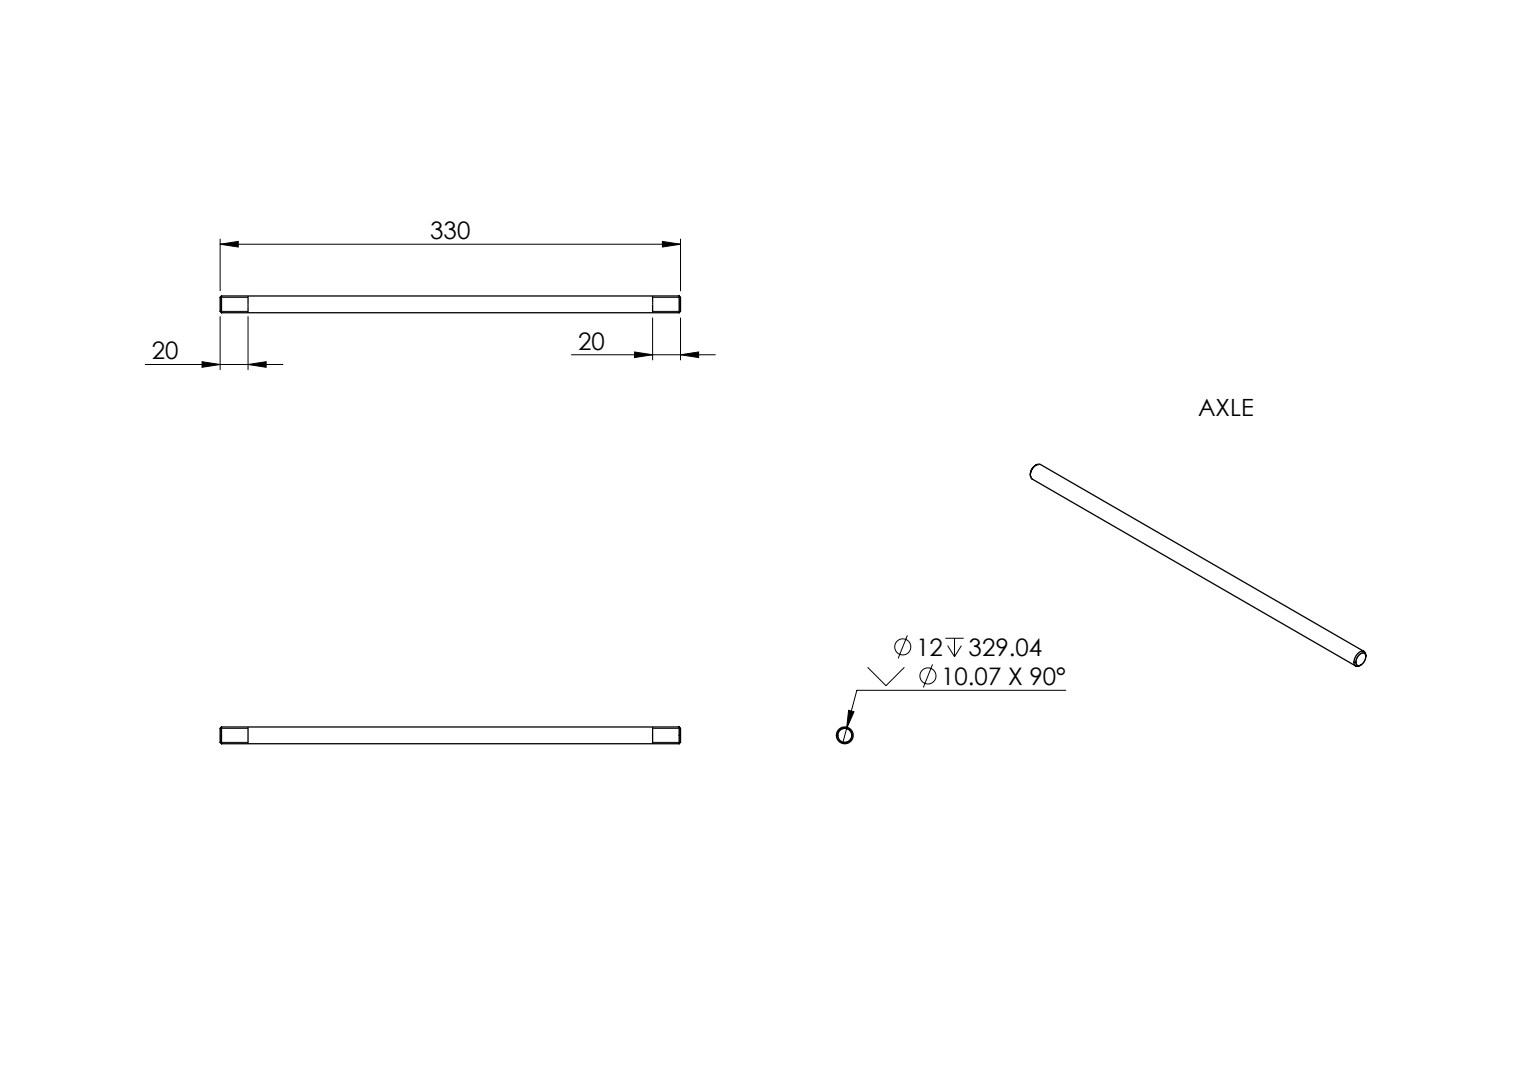
ISO-10303-21;
HEADER;
FILE_DESCRIPTION (('STEP AP214'),
    '1' );
FILE_NAME ('axle.step',
    '2026-10-22T16:49:52',
    ( '' ),
    ( '' ),
    'SwSTEP 2.0',
    'SolidWorks 2026',
    '' );
FILE_SCHEMA (( 'AUTOMOTIVE_DESIGN' ));
ENDSEC;

DATA;
#18=PRODUCT_DEFINITION_SHAPE ( 'NONE', 'NONE',  #4920 ) ;
#47=MANIFOLD_SOLID_BREP ( 'M12 Machine Threads Stud2', #1956 ) ;
#75=ORIENTED_EDGE ( 'NONE', *, *, #1128, .F. ) ;
#88=LINE ( 'NONE', #3399, #4556 ) ;
#132=CARTESIAN_POINT ( 'NONE',  ( 165.0000000000000000, 870.0000000000000000, -5.036000000000040444 ) ) ;
#152=SURFACE_STYLE_USAGE ( .BOTH. , #2636 ) ;
#195=CARTESIAN_POINT ( 'NONE',  ( 165.0000000000000000, 870.0000000000000000, 5.036000000000040444 ) ) ;
#199=CONICAL_SURFACE ( 'NONE', #1255, 5.036000000000040444, 0.7853981633974339571 ) ;
#207=VERTEX_POINT ( 'NONE', #1151 ) ;
#208=AXIS2_PLACEMENT_3D ( 'NONE', #1676, #429, #2877 ) ;
#224=DIRECTION ( 'NONE',  ( 0.000000000000000000, 0.000000000000000000, -1.000000000000000000 ) ) ;
#239=DIRECTION ( 'NONE',  ( -1.000000000000000000, -0.000000000000000000, -0.000000000000000000 ) ) ;
#242=ORIENTED_EDGE ( 'NONE', *, *, #1915, .F. ) ;
#298=CARTESIAN_POINT ( 'NONE',  ( 164.0360000000000014, 870.0000000000000000, -6.000000000000006217 ) ) ;
#302=SHAPE_REPRESENTATION ( 'axle', ( #4154 ), #2055 ) ;
#312=CIRCLE ( 'NONE', #208, 6.000000000000005329 ) ;
#318=SHAPE_REPRESENTATION_RELATIONSHIP ( 'NONE' , 'NONE' ,  #302, #3330 ) ;
#320=ORIENTED_EDGE ( 'NONE', *, *, #1915, .T. ) ;
#323=DIRECTION ( 'NONE',  ( 0.000000000000000000, 0.000000000000000000, 1.000000000000000000 ) ) ;
#339=CARTESIAN_POINT ( 'NONE',  ( 165.0000000000000000, 870.0000000000000000, 0.000000000000000000 ) ) ;
#350=DIRECTION ( 'NONE',  ( -1.000000000000000000, -0.000000000000000000, -0.000000000000000000 ) ) ;
#367=PLANE ( 'NONE',  #841 ) ;
#407=ADVANCED_FACE ( 'NONE', ( #828 ), #1256, .T. ) ;
#424=ORIENTED_EDGE ( 'NONE', *, *, #507, .T. ) ;
#429=DIRECTION ( 'NONE',  ( 1.000000000000000000, -0.000000000000000000, -0.000000000000000000 ) ) ;
#450=( GEOMETRIC_REPRESENTATION_CONTEXT ( 3 ) GLOBAL_UNCERTAINTY_ASSIGNED_CONTEXT ( ( #3198 ) ) GLOBAL_UNIT_ASSIGNED_CONTEXT ( ( #3688, #4189, #3379 ) ) REPRESENTATION_CONTEXT ( 'NONE', 'WORKASPACE' ) );
#463=LINE ( 'NONE', #132, #3357 ) ;
#507=EDGE_CURVE ( 'NONE', #2252, #1603, #88, .T. ) ;
#517=EDGE_CURVE ( 'NONE', #5301, #3270, #463, .T. ) ;
#531=EDGE_CURVE ( 'NONE', #1147, #207, #4577, .T. ) ;
#553=ADVANCED_FACE ( 'NONE', ( #3829 ), #1254, .T. ) ;
#560=DIRECTION ( 'NONE',  ( 0.000000000000000000, 0.000000000000000000, 1.000000000000000000 ) ) ;
#566=AXIS2_PLACEMENT_3D ( 'NONE', #1191, #724, #3740 ) ;
#572=EDGE_LOOP ( 'NONE', ( #2231, #4802, #4354, #3593 ) ) ;
#637=EDGE_LOOP ( 'NONE', ( #743, #2019, #3494, #1929 ) ) ;
#645=ORIENTED_EDGE ( 'NONE', *, *, #531, .T. ) ;
#669=( LENGTH_UNIT ( ) NAMED_UNIT ( * ) SI_UNIT ( .MILLI., .METRE. ) );
#724=DIRECTION ( 'NONE',  ( 1.000000000000000000, -0.000000000000000000, -0.000000000000000000 ) ) ;
#742=EDGE_CURVE ( 'NONE', #1732, #207, #2730, .T. ) ;
#743=ORIENTED_EDGE ( 'NONE', *, *, #4963, .F. ) ;
#763=AXIS2_PLACEMENT_3D ( 'NONE', #3258, #1554, #4883 ) ;
#769=DIRECTION ( 'NONE',  ( 1.000000000000000000, 0.000000000000000000, 0.000000000000000000 ) ) ;
#773=CARTESIAN_POINT ( 'NONE',  ( 165.0000000000000000, 870.0000000000000000, 6.000000000000001776 ) ) ;
#825=VECTOR ( 'NONE', #3989, 999.9999999999998863 ) ;
#828=FACE_OUTER_BOUND ( 'NONE', #1816, .T. ) ;
#841=AXIS2_PLACEMENT_3D ( 'NONE', #5311, #2025, #2001 ) ;
#846=ORIENTED_EDGE ( 'NONE', *, *, #2312, .F. ) ;
#859=EDGE_CURVE ( 'NONE', #1603, #207, #1544, .T. ) ;
#863=ORIENTED_EDGE ( 'NONE', *, *, #517, .T. ) ;
#894=EDGE_CURVE ( 'NONE', #1603, #3270, #4807, .T. ) ;
#896=DIRECTION ( 'NONE',  ( -0.7071067811865577868, 0.000000000000000000, 0.7071067811865373587 ) ) ;
#900=VECTOR ( 'NONE', #3282, 1000.000000000000000 ) ;
#952=ADVANCED_FACE ( 'NONE', ( #3437 ), #2207, .T. ) ;
#968=DIRECTION ( 'NONE',  ( -1.000000000000000000, -0.000000000000000000, -0.000000000000000000 ) ) ;
#996=CARTESIAN_POINT ( 'NONE',  ( 165.0000000000000000, 870.0000000000000000, -5.036000000000040444 ) ) ;
#1018=AXIS2_PLACEMENT_3D ( 'NONE', #2079, #4161, #2987 ) ;
#1028=( NAMED_UNIT ( * ) PLANE_ANGLE_UNIT ( ) SI_UNIT ( $, .RADIAN. ) );
#1031=ORIENTED_EDGE ( 'NONE', *, *, #507, .F. ) ;
#1077=ORIENTED_EDGE ( 'NONE', *, *, #894, .T. ) ;
#1082=DIRECTION ( 'NONE',  ( -1.000000000000000000, -0.000000000000000000, -0.000000000000000000 ) ) ;
#1128=EDGE_CURVE ( 'NONE', #5301, #2252, #4141, .T. ) ;
#1147=VERTEX_POINT ( 'NONE', #2311 ) ;
#1151=CARTESIAN_POINT ( 'NONE',  ( -164.0360000000000014, 870.0000000000000000, 6.000000000000006217 ) ) ;
#1158=FACE_OUTER_BOUND ( 'NONE', #3100, .T. ) ;
#1186=ADVANCED_FACE ( 'NONE', ( #3897 ), #199, .T. ) ;
#1190=MECHANICAL_DESIGN_GEOMETRIC_PRESENTATION_REPRESENTATION('',(#2669),#3462);
#1191=CARTESIAN_POINT ( 'NONE',  ( -165.0000000000000000, 870.0000000000000000, 0.000000000000000000 ) ) ;
#1208=CARTESIAN_POINT ( 'NONE',  ( 165.0000000000000000, 870.0000000000000000, -6.000000000000001776 ) ) ;
#1254=CONICAL_SURFACE ( 'NONE', #3167, 5.036000000000040444, 0.7853981633974339571 ) ;
#1255=AXIS2_PLACEMENT_3D ( 'NONE', #5258, #239, #2255 ) ;
#1256=PLANE ( 'NONE',  #1449 ) ;
#1286=DIRECTION ( 'NONE',  ( 0.000000000000000000, 0.000000000000000000, -1.000000000000000000 ) ) ;
#1371=SURFACE_STYLE_FILL_AREA ( #5086 ) ;
#1449=AXIS2_PLACEMENT_3D ( 'NONE', #339, #4578, #2098 ) ;
#1456=ORIENTED_EDGE ( 'NONE', *, *, #742, .T. ) ;
#1505=CYLINDRICAL_SURFACE ( 'NONE', #4825, 6.000000000000001776 ) ;
#1544=LINE ( 'NONE', #773, #900 ) ;
#1547=DIRECTION ( 'NONE',  ( -1.000000000000000000, -0.000000000000000000, -0.000000000000000000 ) ) ;
#1554=DIRECTION ( 'NONE',  ( -1.000000000000000000, -0.000000000000000000, -0.000000000000000000 ) ) ;
#1558=CARTESIAN_POINT ( 'NONE',  ( -165.0000000000000000, 870.0000000000000000, -5.036000000000040444 ) ) ;
#1603=VERTEX_POINT ( 'NONE', #1961 ) ;
#1676=CARTESIAN_POINT ( 'NONE',  ( -164.0360000000000014, 870.0000000000000000, 0.000000000000000000 ) ) ;
#1681=CARTESIAN_POINT ( 'NONE',  ( 165.0000000000000000, 870.0000000000000000, 0.000000000000000000 ) ) ;
#1705=EDGE_CURVE ( 'NONE', #1732, #2368, #3364, .T. ) ;
#1732=VERTEX_POINT ( 'NONE', #3869 ) ;
#1744=DIRECTION ( 'NONE',  ( 1.000000000000000000, -0.000000000000000000, -0.000000000000000000 ) ) ;
#1795=CARTESIAN_POINT ( 'NONE',  ( -164.0360000000000014, 870.0000000000000000, 0.000000000000000000 ) ) ;
#1814=PRESENTATION_STYLE_ASSIGNMENT (( #152 ) ) ;
#1816=EDGE_LOOP ( 'NONE', ( #242, #75 ) ) ;
#1833=ADVANCED_FACE ( 'NONE', ( #2278 ), #1505, .T. ) ;
#1834=DIRECTION ( 'NONE',  ( 0.7071067811865577868, 0.000000000000000000, -0.7071067811865373587 ) ) ;
#1863=PRODUCT_DEFINITION_FORMATION_WITH_SPECIFIED_SOURCE ( 'ANY', '', #2139, .NOT_KNOWN. ) ;
#1908=FACE_OUTER_BOUND ( 'NONE', #637, .T. ) ;
#1915=EDGE_CURVE ( 'NONE', #2252, #5301, #2306, .T. ) ;
#1929=ORIENTED_EDGE ( 'NONE', *, *, #1992, .T. ) ;
#1955=SHAPE_DEFINITION_REPRESENTATION ( #18, #302 ) ;
#1956=CLOSED_SHELL ( 'NONE', ( #553, #1186, #1833, #3612, #952, #407, #2580, #2460 ) ) ;
#1961=CARTESIAN_POINT ( 'NONE',  ( 164.0360000000000014, 870.0000000000000000, 6.000000000000005329 ) ) ;
#1968=MECHANICAL_DESIGN_GEOMETRIC_PRESENTATION_REPRESENTATION('',(#4732),#450);
#1992=EDGE_CURVE ( 'NONE', #207, #1147, #312, .T. ) ;
#2001=DIRECTION ( 'NONE',  ( 0.000000000000000000, 0.000000000000000000, -1.000000000000000000 ) ) ;
#2019=ORIENTED_EDGE ( 'NONE', *, *, #3681, .T. ) ;
#2025=DIRECTION ( 'NONE',  ( 1.000000000000000000, 0.000000000000000000, 0.000000000000000000 ) ) ;
#2055=( GEOMETRIC_REPRESENTATION_CONTEXT ( 3 ) GLOBAL_UNCERTAINTY_ASSIGNED_CONTEXT ( ( #2829 ) ) GLOBAL_UNIT_ASSIGNED_CONTEXT ( ( #2615, #1028, #3840 ) ) REPRESENTATION_CONTEXT ( 'NONE', 'WORKASPACE' ) );
#2079=CARTESIAN_POINT ( 'NONE',  ( 164.0360000000000014, 870.0000000000000000, 0.000000000000000000 ) ) ;
#2089=CARTESIAN_POINT ( 'NONE',  ( 165.0000000000000000, 870.0000000000000000, 0.000000000000000000 ) ) ;
#2098=DIRECTION ( 'NONE',  ( 0.000000000000000000, 0.000000000000000000, -1.000000000000000000 ) ) ;
#2106=EDGE_LOOP ( 'NONE', ( #320, #863, #3687, #1031 ) ) ;
#2139=PRODUCT ( 'axle', 'axle', '', ( #3254 ) ) ;
#2147=DIRECTION ( 'NONE',  ( 1.000000000000000000, -0.000000000000000000, -0.000000000000000000 ) ) ;
#2156=VECTOR ( 'NONE', #1547, 1000.000000000000000 ) ;
#2197=CARTESIAN_POINT ( 'NONE',  ( -165.0000000000000000, 870.0000000000000000, 0.000000000000000000 ) ) ;
#2207=CONICAL_SURFACE ( 'NONE', #2930, 5.036000000000040444, 0.7853981633974339571 ) ;
#2231=ORIENTED_EDGE ( 'NONE', *, *, #742, .F. ) ;
#2239=CIRCLE ( 'NONE', #1018, 6.000000000000005329 ) ;
#2252=VERTEX_POINT ( 'NONE', #195 ) ;
#2255=DIRECTION ( 'NONE',  ( 0.000000000000000000, 0.000000000000000000, 1.000000000000000000 ) ) ;
#2278=FACE_OUTER_BOUND ( 'NONE', #4065, .T. ) ;
#2306=CIRCLE ( 'NONE', #4646, 5.036000000000040444 ) ;
#2311=CARTESIAN_POINT ( 'NONE',  ( -164.0360000000000014, 870.0000000000000000, -6.000000000000006217 ) ) ;
#2312=EDGE_CURVE ( 'NONE', #2368, #1147, #4398, .T. ) ;
#2316=CARTESIAN_POINT ( 'NONE',  ( -165.0000000000000000, 870.0000000000000000, 5.036000000000040444 ) ) ;
#2341=EDGE_CURVE ( 'NONE', #2368, #1732, #3459, .T. ) ;
#2368=VERTEX_POINT ( 'NONE', #1558 ) ;
#2434=CARTESIAN_POINT ( 'NONE',  ( 0.000000000000000000, 0.000000000000000000, 0.000000000000000000 ) ) ;
#2460=ADVANCED_FACE ( 'NONE', ( #1158 ), #367, .F. ) ;
#2500=AXIS2_PLACEMENT_3D ( 'NONE', #2716, #3940, #224 ) ;
#2580=ADVANCED_FACE ( 'NONE', ( #2692 ), #4738, .T. ) ;
#2615=( LENGTH_UNIT ( ) NAMED_UNIT ( * ) SI_UNIT ( .MILLI., .METRE. ) );
#2618=EDGE_LOOP ( 'NONE', ( #4569, #4690, #424, #3356 ) ) ;
#2636=SURFACE_SIDE_STYLE ('',( #1371 ) ) ;
#2651=AXIS2_PLACEMENT_3D ( 'NONE', #3669, #3249, #4493 ) ;
#2669=STYLED_ITEM ( 'NONE', ( #1814 ), #3330 ) ;
#2692=FACE_OUTER_BOUND ( 'NONE', #572, .T. ) ;
#2716=CARTESIAN_POINT ( 'NONE',  ( -165.0000000000000000, 870.0000000000000000, 0.000000000000000000 ) ) ;
#2730=LINE ( 'NONE', #2316, #825 ) ;
#2780=ORIENTED_EDGE ( 'NONE', *, *, #1705, .F. ) ;
#2786=ORIENTED_EDGE ( 'NONE', *, *, #2341, .T. ) ;
#2829=UNCERTAINTY_MEASURE_WITH_UNIT (LENGTH_MEASURE( 1.000000000000000082E-05 ), #2615, 'distance_accuracy_value', 'NONE');
#2832=( NAMED_UNIT ( * ) SI_UNIT ( $, .STERADIAN. ) SOLID_ANGLE_UNIT ( ) );
#2877=DIRECTION ( 'NONE',  ( 0.000000000000000000, 0.000000000000000000, -1.000000000000000000 ) ) ;
#2885=LINE ( 'NONE', #1208, #2156 ) ;
#2930=AXIS2_PLACEMENT_3D ( 'NONE', #1681, #968, #4255 ) ;
#2951=UNCERTAINTY_MEASURE_WITH_UNIT (LENGTH_MEASURE( 1.000000000000000082E-05 ), #669, 'distance_accuracy_value', 'NONE');
#2987=DIRECTION ( 'NONE',  ( 0.000000000000000000, 0.000000000000000000, 1.000000000000000000 ) ) ;
#3100=EDGE_LOOP ( 'NONE', ( #3537, #2780 ) ) ;
#3167=AXIS2_PLACEMENT_3D ( 'NONE', #5125, #1744, #5074 ) ;
#3197=AXIS2_PLACEMENT_3D ( 'NONE', #1795, #4307, #1286 ) ;
#3198=UNCERTAINTY_MEASURE_WITH_UNIT (LENGTH_MEASURE( 1.000000000000000082E-05 ), #3688, 'distance_accuracy_value', 'NONE');
#3249=DIRECTION ( 'NONE',  ( -1.000000000000000000, -0.000000000000000000, -0.000000000000000000 ) ) ;
#3254=PRODUCT_CONTEXT ( 'NONE', #5160, 'mechanical' ) ;
#3258=CARTESIAN_POINT ( 'NONE',  ( 165.0000000000000000, 870.0000000000000000, 0.000000000000000000 ) ) ;
#3270=VERTEX_POINT ( 'NONE', #298 ) ;
#3282=DIRECTION ( 'NONE',  ( -1.000000000000000000, -0.000000000000000000, -0.000000000000000000 ) ) ;
#3330=ADVANCED_BREP_SHAPE_REPRESENTATION ( '', ( #47, #4154 ), #2055 ) ;
#3356=ORIENTED_EDGE ( 'NONE', *, *, #3681, .F. ) ;
#3357=VECTOR ( 'NONE', #3903, 999.9999999999998863 ) ;
#3364=CIRCLE ( 'NONE', #3793, 5.036000000000040444 ) ;
#3379=( NAMED_UNIT ( * ) SI_UNIT ( $, .STERADIAN. ) SOLID_ANGLE_UNIT ( ) );
#3399=CARTESIAN_POINT ( 'NONE',  ( 165.0000000000000000, 870.0000000000000000, 5.036000000000040444 ) ) ;
#3437=FACE_OUTER_BOUND ( 'NONE', #2618, .T. ) ;
#3459=CIRCLE ( 'NONE', #566, 5.036000000000040444 ) ;
#3462=( GEOMETRIC_REPRESENTATION_CONTEXT ( 3 ) GLOBAL_UNCERTAINTY_ASSIGNED_CONTEXT ( ( #2951 ) ) GLOBAL_UNIT_ASSIGNED_CONTEXT ( ( #669, #4801, #2832 ) ) REPRESENTATION_CONTEXT ( 'NONE', 'WORKASPACE' ) );
#3494=ORIENTED_EDGE ( 'NONE', *, *, #859, .T. ) ;
#3511=CARTESIAN_POINT ( 'NONE',  ( 165.0000000000000000, 870.0000000000000000, 0.000000000000000000 ) ) ;
#3534=VECTOR ( 'NONE', #1834, 999.9999999999998863 ) ;
#3537=ORIENTED_EDGE ( 'NONE', *, *, #2341, .F. ) ;
#3593=ORIENTED_EDGE ( 'NONE', *, *, #1992, .F. ) ;
#3612=ADVANCED_FACE ( 'NONE', ( #1908 ), #5274, .T. ) ;
#3669=CARTESIAN_POINT ( 'NONE',  ( 164.0360000000000014, 870.0000000000000000, 0.000000000000000000 ) ) ;
#3681=EDGE_CURVE ( 'NONE', #3270, #1603, #2239, .T. ) ;
#3687=ORIENTED_EDGE ( 'NONE', *, *, #894, .F. ) ;
#3688=( LENGTH_UNIT ( ) NAMED_UNIT ( * ) SI_UNIT ( .MILLI., .METRE. ) );
#3740=DIRECTION ( 'NONE',  ( 0.000000000000000000, 0.000000000000000000, -1.000000000000000000 ) ) ;
#3793=AXIS2_PLACEMENT_3D ( 'NONE', #2197, #2147, #5089 ) ;
#3815=ORIENTED_EDGE ( 'NONE', *, *, #531, .F. ) ;
#3829=FACE_OUTER_BOUND ( 'NONE', #3996, .T. ) ;
#3840=( NAMED_UNIT ( * ) SI_UNIT ( $, .STERADIAN. ) SOLID_ANGLE_UNIT ( ) );
#3869=CARTESIAN_POINT ( 'NONE',  ( -165.0000000000000000, 870.0000000000000000, 5.036000000000040444 ) ) ;
#3897=FACE_OUTER_BOUND ( 'NONE', #2106, .T. ) ;
#3903=DIRECTION ( 'NONE',  ( -0.7071067811865577868, 8.659560562354808366E-17, -0.7071067811865373587 ) ) ;
#3918=CARTESIAN_POINT ( 'NONE',  ( -165.0000000000000000, 870.0000000000000000, -5.036000000000040444 ) ) ;
#3940=DIRECTION ( 'NONE',  ( 1.000000000000000000, -0.000000000000000000, -0.000000000000000000 ) ) ;
#3950=DIRECTION ( 'NONE',  ( 0.000000000000000000, 0.000000000000000000, 1.000000000000000000 ) ) ;
#3952=CARTESIAN_POINT ( 'NONE',  ( 165.0000000000000000, 870.0000000000000000, 0.000000000000000000 ) ) ;
#3989=DIRECTION ( 'NONE',  ( 0.7071067811865577868, 8.659560562354808366E-17, 0.7071067811865373587 ) ) ;
#3996=EDGE_LOOP ( 'NONE', ( #2786, #1456, #3815, #846 ) ) ;
#4065=EDGE_LOOP ( 'NONE', ( #1077, #5133, #645, #4711 ) ) ;
#4141=CIRCLE ( 'NONE', #5167, 5.036000000000040444 ) ;
#4154=AXIS2_PLACEMENT_3D ( 'NONE', #2434, #5290, #769 ) ;
#4161=DIRECTION ( 'NONE',  ( -1.000000000000000000, -0.000000000000000000, -0.000000000000000000 ) ) ;
#4189=( NAMED_UNIT ( * ) PLANE_ANGLE_UNIT ( ) SI_UNIT ( $, .RADIAN. ) );
#4255=DIRECTION ( 'NONE',  ( 0.000000000000000000, 0.000000000000000000, 1.000000000000000000 ) ) ;
#4307=DIRECTION ( 'NONE',  ( 1.000000000000000000, -0.000000000000000000, -0.000000000000000000 ) ) ;
#4354=ORIENTED_EDGE ( 'NONE', *, *, #2312, .T. ) ;
#4398=LINE ( 'NONE', #3918, #3534 ) ;
#4493=DIRECTION ( 'NONE',  ( 0.000000000000000000, 0.000000000000000000, 1.000000000000000000 ) ) ;
#4556=VECTOR ( 'NONE', #896, 999.9999999999998863 ) ;
#4569=ORIENTED_EDGE ( 'NONE', *, *, #517, .F. ) ;
#4577=CIRCLE ( 'NONE', #3197, 6.000000000000005329 ) ;
#4578=DIRECTION ( 'NONE',  ( 1.000000000000000000, 0.000000000000000000, 0.000000000000000000 ) ) ;
#4646=AXIS2_PLACEMENT_3D ( 'NONE', #2089, #350, #323 ) ;
#4648=COLOUR_RGB ( '',0.8941176470588234615, 0.8941176470588234615, 0.8941176470588234615 ) ;
#4690=ORIENTED_EDGE ( 'NONE', *, *, #1128, .T. ) ;
#4711=ORIENTED_EDGE ( 'NONE', *, *, #859, .F. ) ;
#4732=STYLED_ITEM('',(#5426),#47);
#4738=CONICAL_SURFACE ( 'NONE', #2500, 5.036000000000040444, 0.7853981633974339571 ) ;
#4768=APPLICATION_CONTEXT ( 'automotive_design' ) ;
#4801=( NAMED_UNIT ( * ) PLANE_ANGLE_UNIT ( ) SI_UNIT ( $, .RADIAN. ) );
#4802=ORIENTED_EDGE ( 'NONE', *, *, #1705, .T. ) ;
#4807=CIRCLE ( 'NONE', #2651, 6.000000000000005329 ) ;
#4825=AXIS2_PLACEMENT_3D ( 'NONE', #3511, #5226, #3950 ) ;
#4883=DIRECTION ( 'NONE',  ( 0.000000000000000000, 0.000000000000000000, 1.000000000000000000 ) ) ;
#4920=PRODUCT_DEFINITION ( 'UNKNOWN', '', #1863, #5334 ) ;
#4963=EDGE_CURVE ( 'NONE', #3270, #1147, #2885, .T. ) ;
#5074=DIRECTION ( 'NONE',  ( 0.000000000000000000, 0.000000000000000000, -1.000000000000000000 ) ) ;
#5086=FILL_AREA_STYLE ('',( #5116 ) ) ;
#5089=DIRECTION ( 'NONE',  ( 0.000000000000000000, 0.000000000000000000, -1.000000000000000000 ) ) ;
#5116=FILL_AREA_STYLE_COLOUR ( '', #4648 ) ;
#5125=CARTESIAN_POINT ( 'NONE',  ( -165.0000000000000000, 870.0000000000000000, 0.000000000000000000 ) ) ;
#5133=ORIENTED_EDGE ( 'NONE', *, *, #4963, .T. ) ;
#5160=APPLICATION_CONTEXT ( 'automotive_design' ) ;
#5167=AXIS2_PLACEMENT_3D ( 'NONE', #3952, #1082, #560 ) ;
#5226=DIRECTION ( 'NONE',  ( -1.000000000000000000, -0.000000000000000000, -0.000000000000000000 ) ) ;
#5258=CARTESIAN_POINT ( 'NONE',  ( 165.0000000000000000, 870.0000000000000000, 0.000000000000000000 ) ) ;
#5274=CYLINDRICAL_SURFACE ( 'NONE', #763, 6.000000000000001776 ) ;
#5290=DIRECTION ( 'NONE',  ( 0.000000000000000000, 0.000000000000000000, 1.000000000000000000 ) ) ;
#5301=VERTEX_POINT ( 'NONE', #996 ) ;
#5311=CARTESIAN_POINT ( 'NONE',  ( -165.0000000000000000, 870.0000000000000000, 0.000000000000000000 ) ) ;
#5334=PRODUCT_DEFINITION_CONTEXT ( 'detailed design', #4768, 'design' ) ;
#5420=COLOUR_RGB('Grey',0.48,0.52,0.57);
#5421=FILL_AREA_STYLE_COLOUR('',#5420);
#5422=FILL_AREA_STYLE('',(#5421));
#5423=SURFACE_STYLE_FILL_AREA(#5422);
#5424=SURFACE_SIDE_STYLE('',(#5423));
#5425=SURFACE_STYLE_USAGE(.BOTH.,#5424);
#5426=PRESENTATION_STYLE_ASSIGNMENT((#5425));
ENDSEC;
END-ISO-10303-21;
